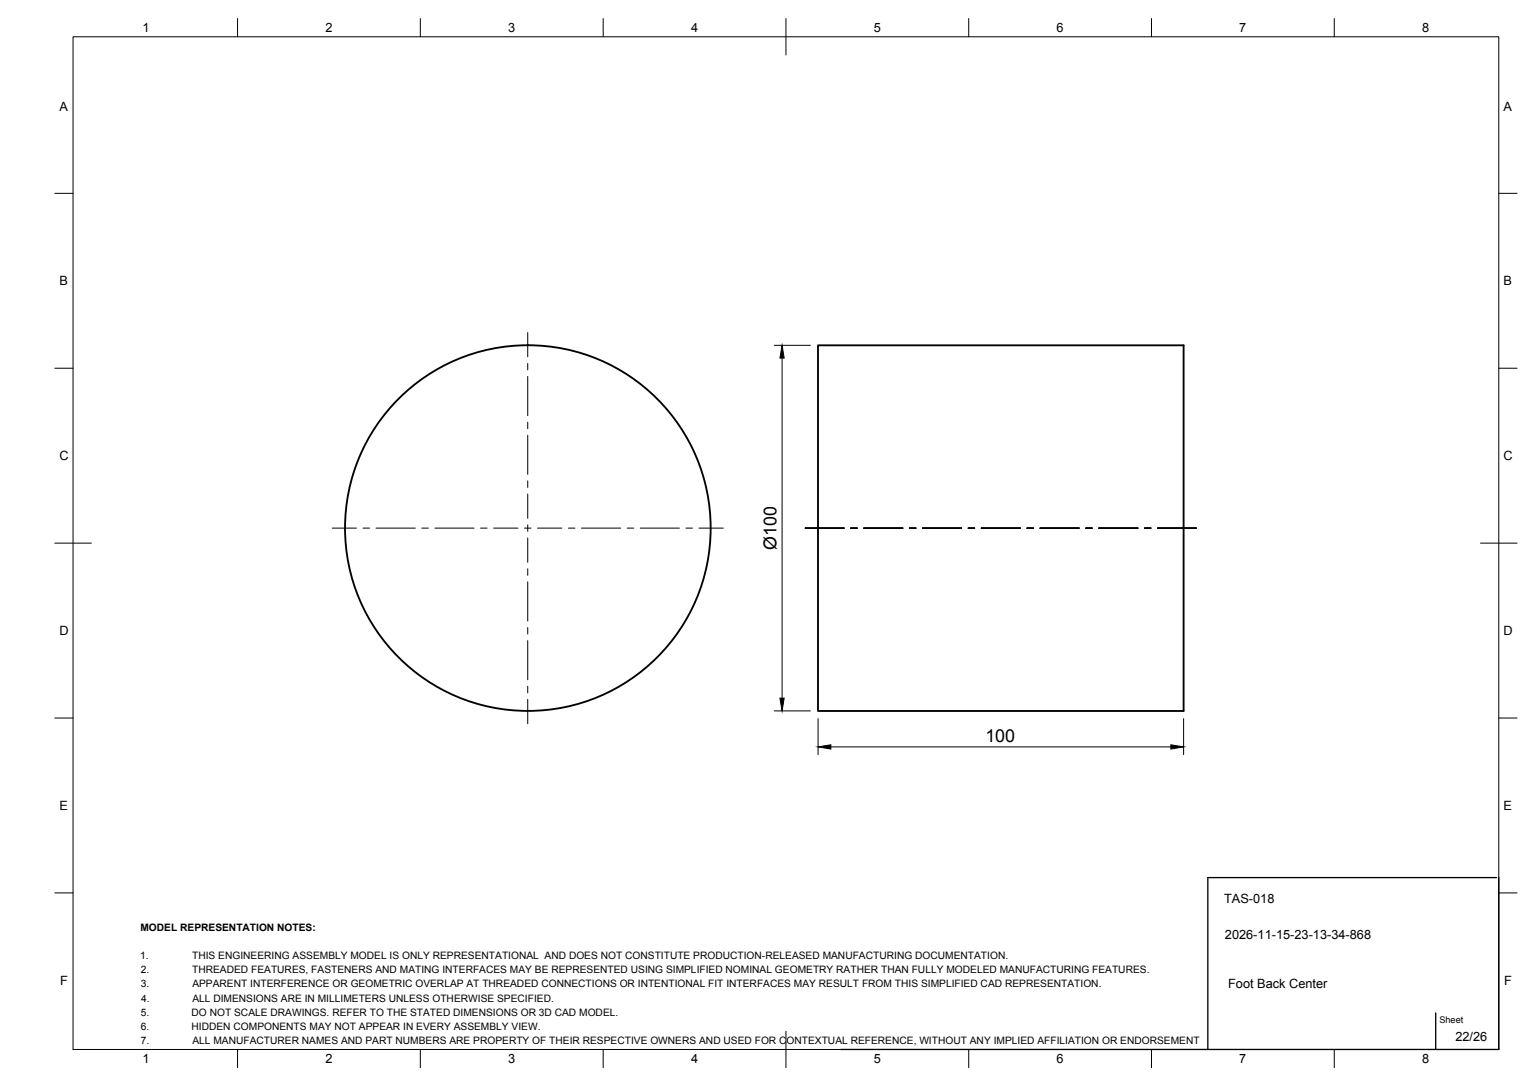
ISO-10303-21;
HEADER;
/* Generated by software containing ST-Developer
 * from STEP Tools, Inc. (www.steptools.com) 
 */

FILE_DESCRIPTION(
/* description */ (''),
/* implementation_level */ '2;1');

FILE_NAME(
/* name */ 'Foot Back Center.step',
/* time_stamp */ '2026-11-15T15:17:57-08:00',
/* author */ (''),
/* organization */ (''),
/* preprocessor_version */ 'ST-DEVELOPER v20.2',
/* originating_system */ 'Autodesk Translation Framework v15.17.0.0',
/* authorisation */ '');

FILE_SCHEMA (('AUTOMOTIVE_DESIGN { 1 0 10303 214 3 1 1 }'));
ENDSEC;

DATA;
#10=MECHANICAL_DESIGN_GEOMETRIC_PRESENTATION_REPRESENTATION('',(#197),#3723);
#21=CIRCLE('',#2454,1.96850393700787);
#22=CIRCLE('',#2455,1.96850393700787);
#28=CYLINDRICAL_SURFACE('',#2453,1.96850393700787);
#149=SHAPE_REPRESENTATION_RELATIONSHIP('SRR','None',#3830,#173);
#173=ADVANCED_BREP_SHAPE_REPRESENTATION('',(#221),#3719);
#197=STYLED_ITEM('',(#3945),#221);
#221=MANIFOLD_SOLID_BREP('Body1',#2045);
#330=FACE_OUTER_BOUND('',#456,.T.);
#331=FACE_OUTER_BOUND('',#457,.T.);
#332=FACE_OUTER_BOUND('',#458,.T.);
#456=EDGE_LOOP('',(#1701,#1702,#1703,#1704));
#457=EDGE_LOOP('',(#1705));
#458=EDGE_LOOP('',(#1706));
#662=LINE('',#3561,#884);
#884=VECTOR('',#2970,1.96850393700787);
#1051=VERTEX_POINT('',#3558);
#1052=VERTEX_POINT('',#3560);
#1272=EDGE_CURVE('',#1051,#1051,#21,.T.);
#1273=EDGE_CURVE('',#1051,#1052,#662,.T.);
#1274=EDGE_CURVE('',#1052,#1052,#22,.T.);
#1701=ORIENTED_EDGE('',*,*,#1272,.T.);
#1702=ORIENTED_EDGE('',*,*,#1273,.T.);
#1703=ORIENTED_EDGE('',*,*,#1274,.F.);
#1704=ORIENTED_EDGE('',*,*,#1273,.F.);
#1705=ORIENTED_EDGE('',*,*,#1274,.T.);
#1706=ORIENTED_EDGE('',*,*,#1272,.F.);
#1879=PLANE('',#2456);
#1880=PLANE('',#2457);
#2004=ADVANCED_FACE('',(#330),#28,.T.);
#2005=ADVANCED_FACE('',(#331),#1879,.T.);
#2006=ADVANCED_FACE('',(#332),#1880,.F.);
#2045=CLOSED_SHELL('',(#2004,#2005,#2006));
#2452=AXIS2_PLACEMENT_3D('',#3556,#2964,#2965);
#2453=AXIS2_PLACEMENT_3D('',#3557,#2966,#2967);
#2454=AXIS2_PLACEMENT_3D('',#3559,#2968,#2969);
#2455=AXIS2_PLACEMENT_3D('',#3562,#2971,#2972);
#2456=AXIS2_PLACEMENT_3D('',#3563,#2973,#2974);
#2457=AXIS2_PLACEMENT_3D('',#3564,#2975,#2976);
#2964=DIRECTION('axis',(0.,0.,1.));
#2965=DIRECTION('refdir',(1.,0.,0.));
#2966=DIRECTION('center_axis',(0.,1.,0.));
#2967=DIRECTION('ref_axis',(0.,0.,1.));
#2968=DIRECTION('center_axis',(0.,-1.,0.));
#2969=DIRECTION('ref_axis',(0.,0.,-1.));
#2970=DIRECTION('',(0.,-1.,0.));
#2971=DIRECTION('center_axis',(0.,-1.,0.));
#2972=DIRECTION('ref_axis',(0.,0.,-1.));
#2973=DIRECTION('center_axis',(0.,-1.,0.));
#2974=DIRECTION('ref_axis',(0.,0.,-1.));
#2975=DIRECTION('center_axis',(0.,-1.,0.));
#2976=DIRECTION('ref_axis',(0.,0.,-1.));
#3556=CARTESIAN_POINT('',(0.,0.,0.));
#3557=CARTESIAN_POINT('Origin',(1.31128703695885E-14,-4.91732638859567E-15,
2.36220472440945));
#3558=CARTESIAN_POINT('',(1.31128703695885E-14,3.93700787401574,0.393700787401575));
#3559=CARTESIAN_POINT('Origin',(1.31128703695885E-14,3.93700787401574,2.36220472440945));
#3560=CARTESIAN_POINT('',(1.31128703695885E-14,-4.91732638859567E-15,0.393700787401575));
#3561=CARTESIAN_POINT('',(1.28717981650319E-14,-4.91732638859567E-15,0.393700787401575));
#3562=CARTESIAN_POINT('Origin',(1.31128703695885E-14,-4.91732638859567E-15,
2.36220472440945));
#3563=CARTESIAN_POINT('Origin',(1.31128703695885E-14,-4.91732638859567E-15,
2.36220472440945));
#3564=CARTESIAN_POINT('Origin',(1.31128703695885E-14,3.93700787401574,2.36220472440945));
#3692=UNCERTAINTY_MEASURE_WITH_UNIT(LENGTH_MEASURE(0.000393700787401575),
#3725,'DISTANCE_ACCURACY_VALUE',
'Maximum model space distance between geometric entities at asserted c
onnectivities');
#3696=UNCERTAINTY_MEASURE_WITH_UNIT(LENGTH_MEASURE(0.000393700787401575),
#3725,'DISTANCE_ACCURACY_VALUE',
'Maximum model space distance between geometric entities at asserted c
onnectivities');
#3719=(
GEOMETRIC_REPRESENTATION_CONTEXT(3)
GLOBAL_UNCERTAINTY_ASSIGNED_CONTEXT((#3692))
GLOBAL_UNIT_ASSIGNED_CONTEXT((#3725,#3729,#3730))
REPRESENTATION_CONTEXT('','3D')
);
#3723=(
GEOMETRIC_REPRESENTATION_CONTEXT(3)
GLOBAL_UNCERTAINTY_ASSIGNED_CONTEXT((#3696))
GLOBAL_UNIT_ASSIGNED_CONTEXT((#3725,#3729,#3730))
REPRESENTATION_CONTEXT('','3D')
);
#3724=DIMENSIONAL_EXPONENTS(1.,0.,0.,0.,0.,0.,0.);
#3725=(
CONVERSION_BASED_UNIT('inch',#3728)
LENGTH_UNIT()
NAMED_UNIT(#3724)
);
#3726=(
LENGTH_UNIT()
NAMED_UNIT(*)
SI_UNIT(.MILLI.,.METRE.)
);
#3728=LENGTH_MEASURE_WITH_UNIT(LENGTH_MEASURE(25.4),#3726);
#3729=(
NAMED_UNIT(*)
PLANE_ANGLE_UNIT()
SI_UNIT($,.RADIAN.)
);
#3730=(
NAMED_UNIT(*)
SI_UNIT($,.STERADIAN.)
SOLID_ANGLE_UNIT()
);
#3753=SHAPE_DEFINITION_REPRESENTATION(#3780,#3830);
#3780=PRODUCT_DEFINITION_SHAPE('',$,#3857);
#3830=SHAPE_REPRESENTATION('',(#2452),#3719);
#3834=PRODUCT_DEFINITION_CONTEXT('part definition',#3914,'design');
#3857=PRODUCT_DEFINITION('2026-11-15-23-13-34-868','Foot Back Center',#3883,
#3834);
#3883=PRODUCT_DEFINITION_FORMATION('',$,#3938);
#3914=APPLICATION_CONTEXT(
'Core Data for Automotive Mechanical Design Process');
#3915=PRODUCT_CONTEXT('part definition',#3914,'mechanical');
#3938=PRODUCT('2026-11-15-23-13-34-868','Foot Back Center',$,(#3915));
#3945=PRESENTATION_STYLE_ASSIGNMENT((#3953));
#3953=SURFACE_STYLE_USAGE(.BOTH.,#3961);
#3961=SURFACE_SIDE_STYLE('',(#3969));
#3969=SURFACE_STYLE_FILL_AREA(#3977);
#3977=FILL_AREA_STYLE('Black',(#3985));
#3985=FILL_AREA_STYLE_COLOUR('Black',#3993);
#3993=COLOUR_RGB('Black',0.0784313725490196,0.0784313725490196,0.0784313725490196);
ENDSEC;
END-ISO-10303-21;
